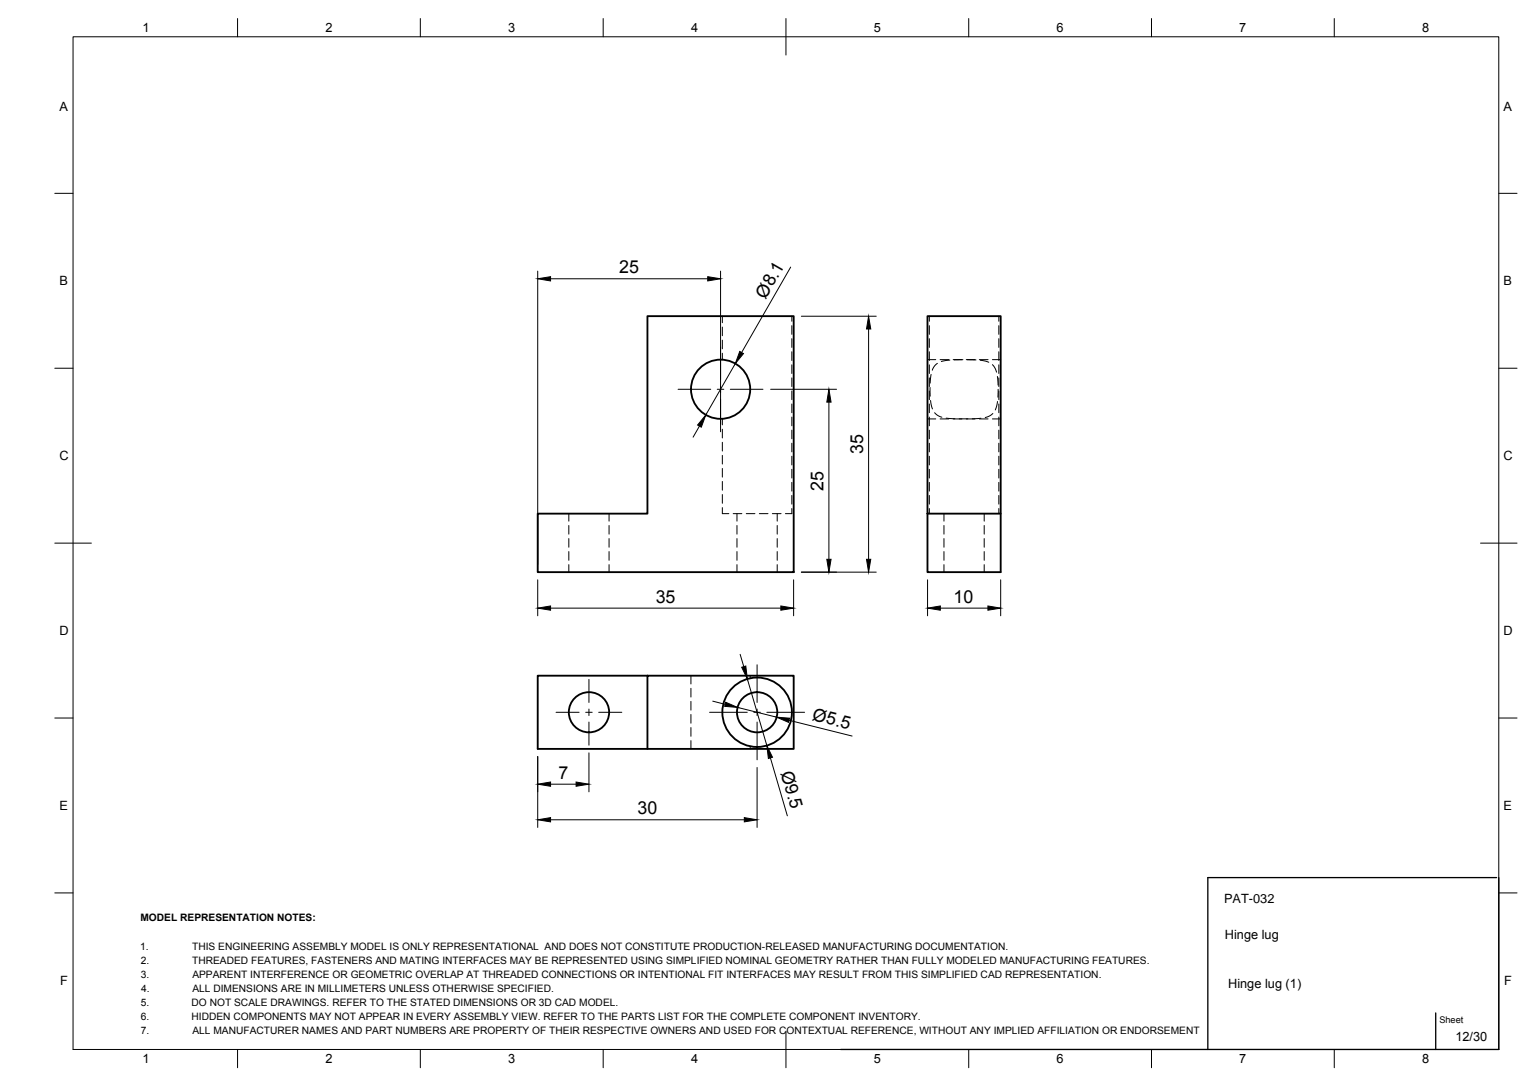
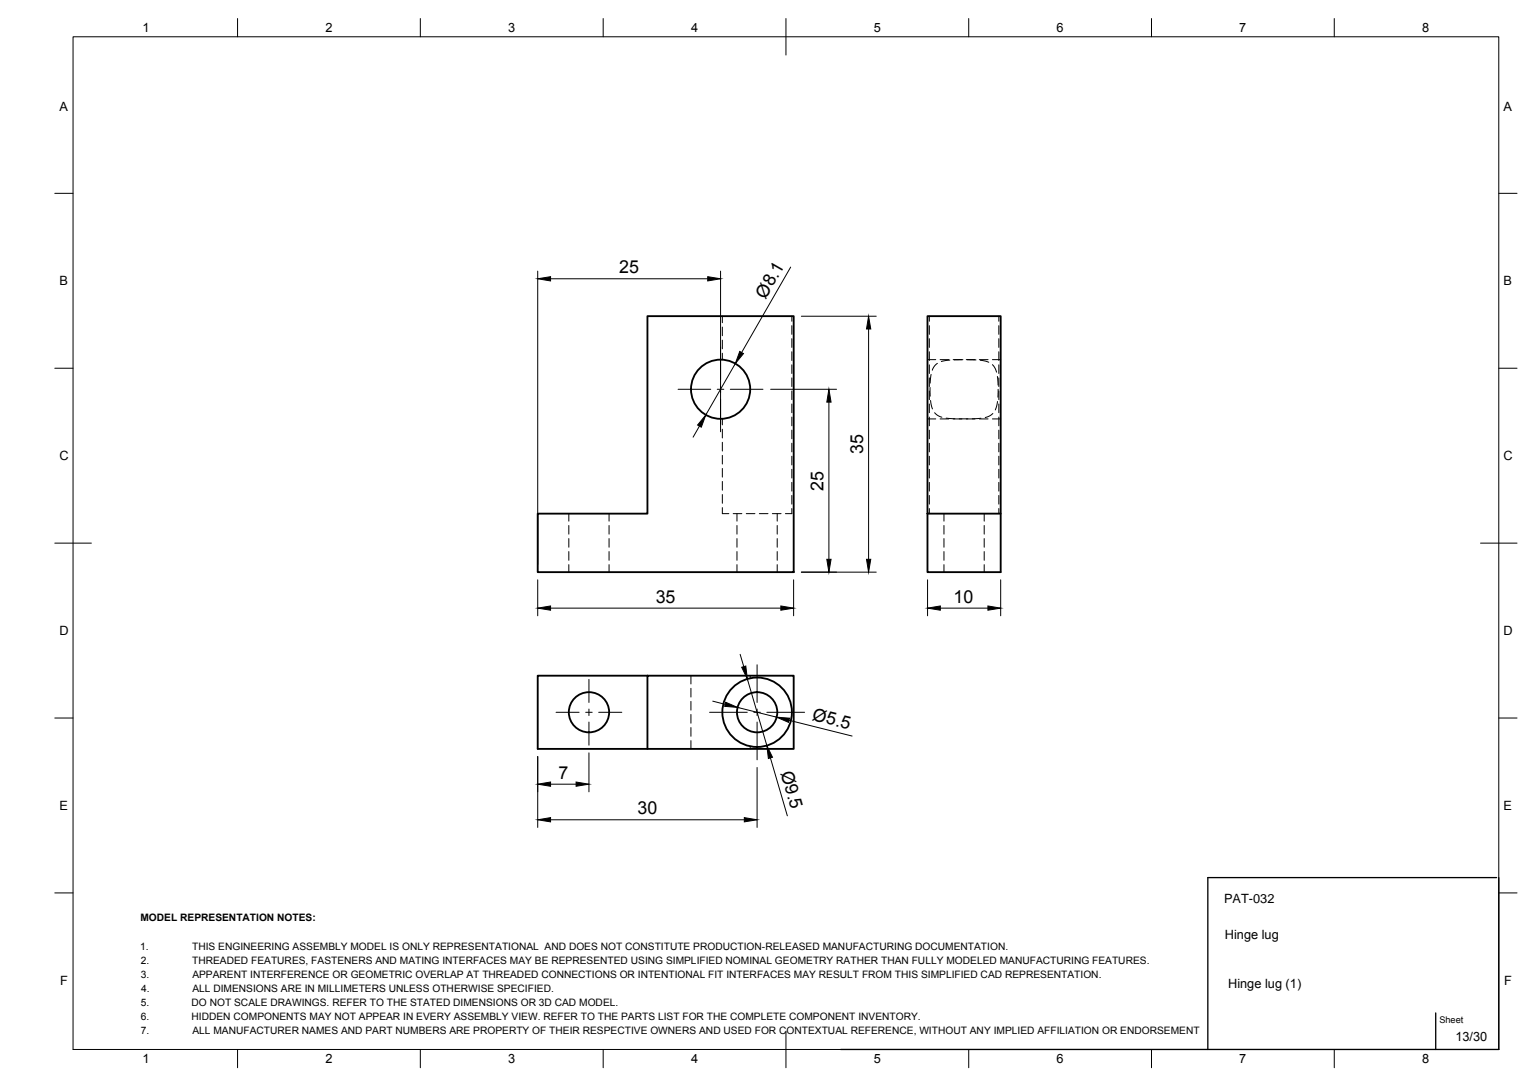
ISO-10303-21;
HEADER;
/* Generated by software containing ST-Developer
 * from STEP Tools, Inc. (www.steptools.com) 
 */

FILE_DESCRIPTION(
/* description */ ('Drill jig with bushing plate'),
/* implementation_level */ '2;1');

FILE_NAME(
/* name */ 'Hinge lug.step',
/* time_stamp */ '2026-10-27T10:51:08-07:00',
/* author */ (''),
/* organization */ (''),
/* preprocessor_version */ 'ST-DEVELOPER v20.2',
/* originating_system */ 'Autodesk Translation Framework v15.17.0.0',
/* authorisation */ '');

FILE_SCHEMA (('AUTOMOTIVE_DESIGN { 1 0 10303 214 3 1 1 }'));
ENDSEC;

DATA;
#10=MECHANICAL_DESIGN_GEOMETRIC_PRESENTATION_REPRESENTATION('',(#230),#6638);
#173=B_SPLINE_CURVE_WITH_KNOTS('',3,(#5774,#5775,#5776,#5777,#5778,#5779,
#5780,#5781,#5782,#5783,#5784,#5785,#5786,#5787,#5788,#5789,#5790,#5791,
#5792,#5793,#5794,#5795,#5796,#5797,#5798,#5799,#5800,#5801,#5802,#5803,
#5804,#5805,#5806,#5807,#5808,#5809,#5810,#5811,#5812,#5813,#5814,#5815,
#5816,#5817,#5818,#5819,#5820,#5821,#5822,#5823),.UNSPECIFIED.,.T.,.F.,
(4,2,2,2,2,2,2,2,2,2,2,2,2,2,2,2,2,2,2,2,2,2,2,2,4),(0.,0.177519856988816,
0.355039713977633,0.436196019741432,0.517352325505232,0.678532215702782,
0.839712105900332,1.00089199609788,1.16207188629543,1.24322819205923,1.32438449782303,
1.50190435481185,1.67942421180066,1.85694406878948,2.0344639257783,2.1156202315421,
2.1967765373059,2.35795642750345,2.519136317701,2.68031620789855,2.8414960980961,
2.9226524038599,3.0038087096237,3.18132856661251,3.35884842360133),
 .UNSPECIFIED.);
#182=SHAPE_REPRESENTATION_RELATIONSHIP('SRR','None',#6746,#206);
#206=ADVANCED_BREP_SHAPE_REPRESENTATION('',(#254),#6619);
#230=STYLED_ITEM('',(#6957),#254);
#254=MANIFOLD_SOLID_BREP('Body1',#3597);
#310=FACE_BOUND('',#818,.T.);
#311=FACE_BOUND('',#820,.T.);
#312=FACE_BOUND('',#824,.T.);
#313=FACE_BOUND('',#826,.T.);
#314=FACE_BOUND('',#829,.T.);
#315=FACE_BOUND('',#832,.T.);
#316=FACE_BOUND('',#833,.T.);
#317=FACE_BOUND('',#836,.T.);
#318=FACE_BOUND('',#838,.T.);
#405=PLANE('',#4007);
#406=PLANE('',#4017);
#407=PLANE('',#4018);
#408=PLANE('',#4019);
#409=PLANE('',#4020);
#410=PLANE('',#4021);
#411=PLANE('',#4022);
#412=PLANE('',#4023);
#413=PLANE('',#4024);
#562=FACE_OUTER_BOUND('',#817,.T.);
#563=FACE_OUTER_BOUND('',#819,.T.);
#564=FACE_OUTER_BOUND('',#821,.T.);
#565=FACE_OUTER_BOUND('',#822,.T.);
#566=FACE_OUTER_BOUND('',#823,.T.);
#567=FACE_OUTER_BOUND('',#825,.T.);
#568=FACE_OUTER_BOUND('',#827,.T.);
#569=FACE_OUTER_BOUND('',#828,.T.);
#570=FACE_OUTER_BOUND('',#830,.T.);
#571=FACE_OUTER_BOUND('',#831,.T.);
#572=FACE_OUTER_BOUND('',#834,.T.);
#573=FACE_OUTER_BOUND('',#835,.T.);
#574=FACE_OUTER_BOUND('',#837,.T.);
#817=EDGE_LOOP('',(#2689,#2690,#2691,#2692));
#818=EDGE_LOOP('',(#2693));
#819=EDGE_LOOP('',(#2694));
#820=EDGE_LOOP('',(#2695));
#821=EDGE_LOOP('',(#2696,#2697,#2698,#2699));
#822=EDGE_LOOP('',(#2700,#2701,#2702,#2703));
#823=EDGE_LOOP('',(#2704,#2705,#2706,#2707));
#824=EDGE_LOOP('',(#2708));
#825=EDGE_LOOP('',(#2709,#2710,#2711,#2712));
#826=EDGE_LOOP('',(#2713));
#827=EDGE_LOOP('',(#2714,#2715,#2716,#2717));
#828=EDGE_LOOP('',(#2718,#2719,#2720,#2721));
#829=EDGE_LOOP('',(#2722));
#830=EDGE_LOOP('',(#2723,#2724,#2725,#2726));
#831=EDGE_LOOP('',(#2727,#2728,#2729,#2730));
#832=EDGE_LOOP('',(#2731));
#833=EDGE_LOOP('',(#2732));
#834=EDGE_LOOP('',(#2733,#2734,#2735,#2736));
#835=EDGE_LOOP('',(#2737,#2738,#2739,#2740,#2741,#2742));
#836=EDGE_LOOP('',(#2743));
#837=EDGE_LOOP('',(#2744,#2745,#2746,#2747,#2748,#2749));
#838=EDGE_LOOP('',(#2750));
#1104=LINE('',#5771,#1365);
#1105=LINE('',#5830,#1366);
#1106=LINE('',#5835,#1367);
#1107=LINE('',#5841,#1368);
#1108=LINE('',#5846,#1369);
#1109=LINE('',#5848,#1370);
#1110=LINE('',#5850,#1371);
#1111=LINE('',#5851,#1372);
#1112=LINE('',#5854,#1373);
#1113=LINE('',#5856,#1374);
#1114=LINE('',#5857,#1375);
#1115=LINE('',#5860,#1376);
#1116=LINE('',#5862,#1377);
#1117=LINE('',#5863,#1378);
#1118=LINE('',#5866,#1379);
#1119=LINE('',#5868,#1380);
#1120=LINE('',#5869,#1381);
#1121=LINE('',#5872,#1382);
#1122=LINE('',#5874,#1383);
#1123=LINE('',#5875,#1384);
#1124=LINE('',#5877,#1385);
#1125=LINE('',#5878,#1386);
#1365=VECTOR('',#4653,0.475);
#1366=VECTOR('',#4664,0.275);
#1367=VECTOR('',#4669,0.275);
#1368=VECTOR('',#4676,0.405);
#1369=VECTOR('',#4681,1.);
#1370=VECTOR('',#4682,1.);
#1371=VECTOR('',#4683,1.);
#1372=VECTOR('',#4684,1.);
#1373=VECTOR('',#4687,1.);
#1374=VECTOR('',#4688,1.);
#1375=VECTOR('',#4689,1.);
#1376=VECTOR('',#4692,1.);
#1377=VECTOR('',#4693,1.);
#1378=VECTOR('',#4694,1.);
#1379=VECTOR('',#4697,1.);
#1380=VECTOR('',#4698,1.);
#1381=VECTOR('',#4699,1.);
#1382=VECTOR('',#4702,1.);
#1383=VECTOR('',#4703,1.);
#1384=VECTOR('',#4704,1.);
#1385=VECTOR('',#4707,1.);
#1386=VECTOR('',#4708,1.);
#1604=CIRCLE('',#4005,0.475);
#1605=CIRCLE('',#4006,0.475);
#1606=CIRCLE('',#4008,0.275);
#1607=CIRCLE('',#4010,0.275);
#1608=CIRCLE('',#4012,0.275);
#1609=CIRCLE('',#4013,0.275);
#1610=CIRCLE('',#4015,0.405);
#1611=CIRCLE('',#4016,0.405);
#1804=VERTEX_POINT('',#5768);
#1805=VERTEX_POINT('',#5770);
#1806=VERTEX_POINT('',#5773);
#1807=VERTEX_POINT('',#5825);
#1808=VERTEX_POINT('',#5828);
#1809=VERTEX_POINT('',#5832);
#1810=VERTEX_POINT('',#5834);
#1811=VERTEX_POINT('',#5838);
#1812=VERTEX_POINT('',#5840);
#1813=VERTEX_POINT('',#5844);
#1814=VERTEX_POINT('',#5845);
#1815=VERTEX_POINT('',#5847);
#1816=VERTEX_POINT('',#5849);
#1817=VERTEX_POINT('',#5853);
#1818=VERTEX_POINT('',#5855);
#1819=VERTEX_POINT('',#5859);
#1820=VERTEX_POINT('',#5861);
#1821=VERTEX_POINT('',#5865);
#1822=VERTEX_POINT('',#5867);
#1823=VERTEX_POINT('',#5871);
#1824=VERTEX_POINT('',#5873);
#2132=EDGE_CURVE('',#1804,#1804,#1604,.T.);
#2133=EDGE_CURVE('',#1804,#1805,#1104,.T.);
#2134=EDGE_CURVE('',#1805,#1805,#1605,.T.);
#2135=EDGE_CURVE('',#1806,#1806,#173,.T.);
#2136=EDGE_CURVE('',#1807,#1807,#1606,.T.);
#2137=EDGE_CURVE('',#1808,#1808,#1607,.T.);
#2138=EDGE_CURVE('',#1808,#1807,#1105,.T.);
#2139=EDGE_CURVE('',#1809,#1809,#1608,.T.);
#2140=EDGE_CURVE('',#1809,#1810,#1106,.T.);
#2141=EDGE_CURVE('',#1810,#1810,#1609,.T.);
#2142=EDGE_CURVE('',#1811,#1811,#1610,.T.);
#2143=EDGE_CURVE('',#1811,#1812,#1107,.T.);
#2144=EDGE_CURVE('',#1812,#1812,#1611,.T.);
#2145=EDGE_CURVE('',#1813,#1814,#1108,.T.);
#2146=EDGE_CURVE('',#1814,#1815,#1109,.T.);
#2147=EDGE_CURVE('',#1816,#1815,#1110,.T.);
#2148=EDGE_CURVE('',#1813,#1816,#1111,.T.);
#2149=EDGE_CURVE('',#1817,#1813,#1112,.T.);
#2150=EDGE_CURVE('',#1818,#1816,#1113,.T.);
#2151=EDGE_CURVE('',#1817,#1818,#1114,.T.);
#2152=EDGE_CURVE('',#1819,#1817,#1115,.T.);
#2153=EDGE_CURVE('',#1820,#1818,#1116,.T.);
#2154=EDGE_CURVE('',#1819,#1820,#1117,.T.);
#2155=EDGE_CURVE('',#1821,#1819,#1118,.T.);
#2156=EDGE_CURVE('',#1822,#1820,#1119,.T.);
#2157=EDGE_CURVE('',#1821,#1822,#1120,.T.);
#2158=EDGE_CURVE('',#1823,#1821,#1121,.T.);
#2159=EDGE_CURVE('',#1824,#1822,#1122,.T.);
#2160=EDGE_CURVE('',#1823,#1824,#1123,.T.);
#2161=EDGE_CURVE('',#1814,#1823,#1124,.T.);
#2162=EDGE_CURVE('',#1815,#1824,#1125,.T.);
#2689=ORIENTED_EDGE('',*,*,#2132,.F.);
#2690=ORIENTED_EDGE('',*,*,#2133,.T.);
#2691=ORIENTED_EDGE('',*,*,#2134,.F.);
#2692=ORIENTED_EDGE('',*,*,#2133,.F.);
#2693=ORIENTED_EDGE('',*,*,#2135,.F.);
#2694=ORIENTED_EDGE('',*,*,#2132,.T.);
#2695=ORIENTED_EDGE('',*,*,#2136,.F.);
#2696=ORIENTED_EDGE('',*,*,#2137,.F.);
#2697=ORIENTED_EDGE('',*,*,#2138,.T.);
#2698=ORIENTED_EDGE('',*,*,#2136,.T.);
#2699=ORIENTED_EDGE('',*,*,#2138,.F.);
#2700=ORIENTED_EDGE('',*,*,#2139,.F.);
#2701=ORIENTED_EDGE('',*,*,#2140,.T.);
#2702=ORIENTED_EDGE('',*,*,#2141,.F.);
#2703=ORIENTED_EDGE('',*,*,#2140,.F.);
#2704=ORIENTED_EDGE('',*,*,#2142,.F.);
#2705=ORIENTED_EDGE('',*,*,#2143,.T.);
#2706=ORIENTED_EDGE('',*,*,#2144,.F.);
#2707=ORIENTED_EDGE('',*,*,#2143,.F.);
#2708=ORIENTED_EDGE('',*,*,#2135,.T.);
#2709=ORIENTED_EDGE('',*,*,#2145,.T.);
#2710=ORIENTED_EDGE('',*,*,#2146,.T.);
#2711=ORIENTED_EDGE('',*,*,#2147,.F.);
#2712=ORIENTED_EDGE('',*,*,#2148,.F.);
#2713=ORIENTED_EDGE('',*,*,#2134,.T.);
#2714=ORIENTED_EDGE('',*,*,#2149,.T.);
#2715=ORIENTED_EDGE('',*,*,#2148,.T.);
#2716=ORIENTED_EDGE('',*,*,#2150,.F.);
#2717=ORIENTED_EDGE('',*,*,#2151,.F.);
#2718=ORIENTED_EDGE('',*,*,#2152,.T.);
#2719=ORIENTED_EDGE('',*,*,#2151,.T.);
#2720=ORIENTED_EDGE('',*,*,#2153,.F.);
#2721=ORIENTED_EDGE('',*,*,#2154,.F.);
#2722=ORIENTED_EDGE('',*,*,#2141,.T.);
#2723=ORIENTED_EDGE('',*,*,#2155,.T.);
#2724=ORIENTED_EDGE('',*,*,#2154,.T.);
#2725=ORIENTED_EDGE('',*,*,#2156,.F.);
#2726=ORIENTED_EDGE('',*,*,#2157,.F.);
#2727=ORIENTED_EDGE('',*,*,#2158,.T.);
#2728=ORIENTED_EDGE('',*,*,#2157,.T.);
#2729=ORIENTED_EDGE('',*,*,#2159,.F.);
#2730=ORIENTED_EDGE('',*,*,#2160,.F.);
#2731=ORIENTED_EDGE('',*,*,#2137,.T.);
#2732=ORIENTED_EDGE('',*,*,#2139,.T.);
#2733=ORIENTED_EDGE('',*,*,#2161,.T.);
#2734=ORIENTED_EDGE('',*,*,#2160,.T.);
#2735=ORIENTED_EDGE('',*,*,#2162,.F.);
#2736=ORIENTED_EDGE('',*,*,#2146,.F.);
#2737=ORIENTED_EDGE('',*,*,#2162,.T.);
#2738=ORIENTED_EDGE('',*,*,#2159,.T.);
#2739=ORIENTED_EDGE('',*,*,#2156,.T.);
#2740=ORIENTED_EDGE('',*,*,#2153,.T.);
#2741=ORIENTED_EDGE('',*,*,#2150,.T.);
#2742=ORIENTED_EDGE('',*,*,#2147,.T.);
#2743=ORIENTED_EDGE('',*,*,#2144,.T.);
#2744=ORIENTED_EDGE('',*,*,#2161,.F.);
#2745=ORIENTED_EDGE('',*,*,#2145,.F.);
#2746=ORIENTED_EDGE('',*,*,#2149,.F.);
#2747=ORIENTED_EDGE('',*,*,#2152,.F.);
#2748=ORIENTED_EDGE('',*,*,#2155,.F.);
#2749=ORIENTED_EDGE('',*,*,#2158,.F.);
#2750=ORIENTED_EDGE('',*,*,#2142,.T.);
#3325=CYLINDRICAL_SURFACE('',#4004,0.475);
#3326=CYLINDRICAL_SURFACE('',#4009,0.275);
#3327=CYLINDRICAL_SURFACE('',#4011,0.275);
#3328=CYLINDRICAL_SURFACE('',#4014,0.405);
#3437=ADVANCED_FACE('',(#562,#310),#3325,.F.);
#3438=ADVANCED_FACE('',(#563,#311),#405,.T.);
#3439=ADVANCED_FACE('',(#564),#3326,.F.);
#3440=ADVANCED_FACE('',(#565),#3327,.F.);
#3441=ADVANCED_FACE('',(#566,#312),#3328,.F.);
#3442=ADVANCED_FACE('',(#567,#313),#406,.T.);
#3443=ADVANCED_FACE('',(#568),#407,.T.);
#3444=ADVANCED_FACE('',(#569,#314),#408,.T.);
#3445=ADVANCED_FACE('',(#570),#409,.T.);
#3446=ADVANCED_FACE('',(#571,#315,#316),#410,.T.);
#3447=ADVANCED_FACE('',(#572),#411,.T.);
#3448=ADVANCED_FACE('',(#573,#317),#412,.T.);
#3449=ADVANCED_FACE('',(#574,#318),#413,.F.);
#3597=CLOSED_SHELL('',(#3437,#3438,#3439,#3440,#3441,#3442,#3443,#3444,
#3445,#3446,#3447,#3448,#3449));
#4003=AXIS2_PLACEMENT_3D('',#5766,#4647,#4648);
#4004=AXIS2_PLACEMENT_3D('',#5767,#4649,#4650);
#4005=AXIS2_PLACEMENT_3D('',#5769,#4651,#4652);
#4006=AXIS2_PLACEMENT_3D('',#5772,#4654,#4655);
#4007=AXIS2_PLACEMENT_3D('',#5824,#4656,#4657);
#4008=AXIS2_PLACEMENT_3D('',#5826,#4658,#4659);
#4009=AXIS2_PLACEMENT_3D('',#5827,#4660,#4661);
#4010=AXIS2_PLACEMENT_3D('',#5829,#4662,#4663);
#4011=AXIS2_PLACEMENT_3D('',#5831,#4665,#4666);
#4012=AXIS2_PLACEMENT_3D('',#5833,#4667,#4668);
#4013=AXIS2_PLACEMENT_3D('',#5836,#4670,#4671);
#4014=AXIS2_PLACEMENT_3D('',#5837,#4672,#4673);
#4015=AXIS2_PLACEMENT_3D('',#5839,#4674,#4675);
#4016=AXIS2_PLACEMENT_3D('',#5842,#4677,#4678);
#4017=AXIS2_PLACEMENT_3D('',#5843,#4679,#4680);
#4018=AXIS2_PLACEMENT_3D('',#5852,#4685,#4686);
#4019=AXIS2_PLACEMENT_3D('',#5858,#4690,#4691);
#4020=AXIS2_PLACEMENT_3D('',#5864,#4695,#4696);
#4021=AXIS2_PLACEMENT_3D('',#5870,#4700,#4701);
#4022=AXIS2_PLACEMENT_3D('',#5876,#4705,#4706);
#4023=AXIS2_PLACEMENT_3D('',#5879,#4709,#4710);
#4024=AXIS2_PLACEMENT_3D('',#5880,#4711,#4712);
#4647=DIRECTION('axis',(0.,0.,1.));
#4648=DIRECTION('refdir',(1.,0.,0.));
#4649=DIRECTION('center_axis',(0.,0.,1.));
#4650=DIRECTION('ref_axis',(1.,0.,0.));
#4651=DIRECTION('center_axis',(0.,0.,1.));
#4652=DIRECTION('ref_axis',(1.,0.,0.));
#4653=DIRECTION('',(0.,0.,1.));
#4654=DIRECTION('center_axis',(0.,0.,-1.));
#4655=DIRECTION('ref_axis',(1.,0.,0.));
#4656=DIRECTION('center_axis',(0.,0.,1.));
#4657=DIRECTION('ref_axis',(1.,0.,0.));
#4658=DIRECTION('center_axis',(0.,0.,1.));
#4659=DIRECTION('ref_axis',(1.,0.,0.));
#4660=DIRECTION('center_axis',(0.,0.,1.));
#4661=DIRECTION('ref_axis',(1.,0.,0.));
#4662=DIRECTION('center_axis',(0.,0.,1.));
#4663=DIRECTION('ref_axis',(1.,0.,0.));
#4664=DIRECTION('',(0.,0.,1.));
#4665=DIRECTION('center_axis',(0.,0.,1.));
#4666=DIRECTION('ref_axis',(1.,0.,0.));
#4667=DIRECTION('center_axis',(0.,0.,1.));
#4668=DIRECTION('ref_axis',(1.,0.,0.));
#4669=DIRECTION('',(0.,0.,1.));
#4670=DIRECTION('center_axis',(0.,0.,-1.));
#4671=DIRECTION('ref_axis',(1.,0.,0.));
#4672=DIRECTION('center_axis',(1.,0.,0.));
#4673=DIRECTION('ref_axis',(0.,0.,-1.));
#4674=DIRECTION('center_axis',(1.,0.,0.));
#4675=DIRECTION('ref_axis',(0.,0.,-1.));
#4676=DIRECTION('',(1.,0.,0.));
#4677=DIRECTION('center_axis',(-1.,0.,0.));
#4678=DIRECTION('ref_axis',(0.,0.,-1.));
#4679=DIRECTION('center_axis',(0.,0.,1.));
#4680=DIRECTION('ref_axis',(0.,-1.,0.));
#4681=DIRECTION('',(0.,-1.,0.));
#4682=DIRECTION('',(1.,0.,0.));
#4683=DIRECTION('',(0.,-1.,0.));
#4684=DIRECTION('',(1.,0.,0.));
#4685=DIRECTION('center_axis',(0.,1.,0.));
#4686=DIRECTION('ref_axis',(0.,0.,1.));
#4687=DIRECTION('',(0.,0.,1.));
#4688=DIRECTION('',(0.,0.,1.));
#4689=DIRECTION('',(1.,0.,0.));
#4690=DIRECTION('center_axis',(0.,0.,1.));
#4691=DIRECTION('ref_axis',(0.,-1.,0.));
#4692=DIRECTION('',(0.,-1.,0.));
#4693=DIRECTION('',(0.,-1.,0.));
#4694=DIRECTION('',(1.,0.,0.));
#4695=DIRECTION('center_axis',(0.,1.,0.));
#4696=DIRECTION('ref_axis',(0.,0.,1.));
#4697=DIRECTION('',(0.,0.,1.));
#4698=DIRECTION('',(0.,0.,1.));
#4699=DIRECTION('',(1.,0.,0.));
#4700=DIRECTION('center_axis',(0.,0.,-1.));
#4701=DIRECTION('ref_axis',(0.,1.,0.));
#4702=DIRECTION('',(0.,1.,0.));
#4703=DIRECTION('',(0.,1.,0.));
#4704=DIRECTION('',(1.,0.,0.));
#4705=DIRECTION('center_axis',(0.,-1.,0.));
#4706=DIRECTION('ref_axis',(0.,0.,-1.));
#4707=DIRECTION('',(0.,0.,-1.));
#4708=DIRECTION('',(0.,0.,-1.));
#4709=DIRECTION('center_axis',(1.,0.,0.));
#4710=DIRECTION('ref_axis',(0.,0.,-1.));
#4711=DIRECTION('center_axis',(1.,0.,0.));
#4712=DIRECTION('ref_axis',(0.,0.,-1.));
#5766=CARTESIAN_POINT('',(0.,0.,0.));
#5767=CARTESIAN_POINT('Origin',(-6.5,-6.5,1.8));
#5768=CARTESIAN_POINT('',(-6.975,-6.5,1.8));
#5769=CARTESIAN_POINT('Origin',(-6.5,-6.5,1.8));
#5770=CARTESIAN_POINT('',(-6.975,-6.5,4.5));
#5771=CARTESIAN_POINT('',(-6.975,-6.5,1.8));
#5772=CARTESIAN_POINT('Origin',(-6.5,-6.5,4.5));
#5773=CARTESIAN_POINT('',(-6.9654030511288,-6.405,3.5));
#5774=CARTESIAN_POINT('Ctrl Pts',(-6.9654030511288,-6.405,3.5));
#5775=CARTESIAN_POINT('Ctrl Pts',(-6.9654030511288,-6.405,3.44082671433706));
#5776=CARTESIAN_POINT('Ctrl Pts',(-6.96319194510978,-6.391162819218,3.3786038562345));
#5777=CARTESIAN_POINT('Ctrl Pts',(-6.9474004570938,-6.33805779261652,3.26878119899199));
#5778=CARTESIAN_POINT('Ctrl Pts',(-6.93296763252909,-6.29875591394082,3.22132213181236));
#5779=CARTESIAN_POINT('Ctrl Pts',(-6.89697744222372,-6.23823300006139,3.17155768103299));
#5780=CARTESIAN_POINT('Ctrl Pts',(-6.88237408148839,-6.2169021926909,3.15715697182391));
#5781=CARTESIAN_POINT('Ctrl Pts',(-6.84782319019902,-6.17538739566531,3.13417605500228));
#5782=CARTESIAN_POINT('Ctrl Pts',(-6.8278469830262,-6.1552757719279,3.12550838237099));
#5783=CARTESIAN_POINT('Ctrl Pts',(-6.76795622589237,-6.10432382827604,3.1070097286502));
#5784=CARTESIAN_POINT('Ctrl Pts',(-6.71846870594364,-6.07437258197005,3.10138466314703));
#5785=CARTESIAN_POINT('Ctrl Pts',(-6.61134072173687,-6.03471454832095,3.09599463066268));
#5786=CARTESIAN_POINT('Ctrl Pts',(-6.55372663006585,-6.025,3.09577234137185));
#5787=CARTESIAN_POINT('Ctrl Pts',(-6.44627336993415,-6.025,3.09577234137185));
#5788=CARTESIAN_POINT('Ctrl Pts',(-6.38865927826313,-6.03471454832095,3.09599463066268));
#5789=CARTESIAN_POINT('Ctrl Pts',(-6.28153129405636,-6.07437258197005,3.10138466314702));
#5790=CARTESIAN_POINT('Ctrl Pts',(-6.23204377410763,-6.10432382827604,3.1070097286502));
#5791=CARTESIAN_POINT('Ctrl Pts',(-6.1721530169738,-6.1552757719279,3.12550838237099));
#5792=CARTESIAN_POINT('Ctrl Pts',(-6.15217680980098,-6.17538739566531,3.13417605500228));
#5793=CARTESIAN_POINT('Ctrl Pts',(-6.11762591851161,-6.2169021926909,3.15715697182391));
#5794=CARTESIAN_POINT('Ctrl Pts',(-6.10302255777628,-6.23823300006139,3.17155768103299));
#5795=CARTESIAN_POINT('Ctrl Pts',(-6.06703236747091,-6.29875591394082,3.22132213181236));
#5796=CARTESIAN_POINT('Ctrl Pts',(-6.0525995429062,-6.33805779261652,3.26878119899199));
#5797=CARTESIAN_POINT('Ctrl Pts',(-6.03680805489022,-6.391162819218,3.3786038562345));
#5798=CARTESIAN_POINT('Ctrl Pts',(-6.0345969488712,-6.405,3.44082671433706));
#5799=CARTESIAN_POINT('Ctrl Pts',(-6.0345969488712,-6.405,3.55917328566294));
#5800=CARTESIAN_POINT('Ctrl Pts',(-6.03680805489022,-6.391162819218,3.6213961437655));
#5801=CARTESIAN_POINT('Ctrl Pts',(-6.0525995429062,-6.33805779261652,3.73121880100801));
#5802=CARTESIAN_POINT('Ctrl Pts',(-6.06703236747091,-6.29875591394082,3.77867786818764));
#5803=CARTESIAN_POINT('Ctrl Pts',(-6.10302255777628,-6.23823300006139,3.82844231896701));
#5804=CARTESIAN_POINT('Ctrl Pts',(-6.1176259185116,-6.2169021926909,3.84284302817609));
#5805=CARTESIAN_POINT('Ctrl Pts',(-6.15217680980098,-6.17538739566531,3.86582394499772));
#5806=CARTESIAN_POINT('Ctrl Pts',(-6.1721530169738,-6.1552757719279,3.87449161762901));
#5807=CARTESIAN_POINT('Ctrl Pts',(-6.23204377410763,-6.10432382827604,3.8929902713498));
#5808=CARTESIAN_POINT('Ctrl Pts',(-6.28153129405636,-6.07437258197005,3.89861533685297));
#5809=CARTESIAN_POINT('Ctrl Pts',(-6.38865927826313,-6.03471454832095,3.90400536933732));
#5810=CARTESIAN_POINT('Ctrl Pts',(-6.44627336993415,-6.025,3.90422765862815));
#5811=CARTESIAN_POINT('Ctrl Pts',(-6.55372663006585,-6.025,3.90422765862815));
#5812=CARTESIAN_POINT('Ctrl Pts',(-6.61134072173687,-6.03471454832095,3.90400536933732));
#5813=CARTESIAN_POINT('Ctrl Pts',(-6.71846870594364,-6.07437258197005,3.89861533685297));
#5814=CARTESIAN_POINT('Ctrl Pts',(-6.76795622589237,-6.10432382827604,3.8929902713498));
#5815=CARTESIAN_POINT('Ctrl Pts',(-6.8278469830262,-6.1552757719279,3.87449161762901));
#5816=CARTESIAN_POINT('Ctrl Pts',(-6.84782319019902,-6.17538739566531,3.86582394499772));
#5817=CARTESIAN_POINT('Ctrl Pts',(-6.8823740814884,-6.21690219269089,3.84284302817609));
#5818=CARTESIAN_POINT('Ctrl Pts',(-6.89697744222372,-6.23823300006139,3.82844231896701));
#5819=CARTESIAN_POINT('Ctrl Pts',(-6.93296763252909,-6.29875591394082,3.77867786818764));
#5820=CARTESIAN_POINT('Ctrl Pts',(-6.9474004570938,-6.33805779261652,3.73121880100801));
#5821=CARTESIAN_POINT('Ctrl Pts',(-6.96319194510978,-6.391162819218,3.6213961437655));
#5822=CARTESIAN_POINT('Ctrl Pts',(-6.9654030511288,-6.405,3.55917328566294));
#5823=CARTESIAN_POINT('Ctrl Pts',(-6.9654030511288,-6.405,3.5));
#5824=CARTESIAN_POINT('Origin',(-6.5,-6.5,1.8));
#5825=CARTESIAN_POINT('',(-6.775,-6.5,1.8));
#5826=CARTESIAN_POINT('Origin',(-6.5,-6.5,1.8));
#5827=CARTESIAN_POINT('Origin',(-6.5,-6.5,0.9));
#5828=CARTESIAN_POINT('',(-6.775,-6.5,1.));
#5829=CARTESIAN_POINT('Origin',(-6.5,-6.5,1.));
#5830=CARTESIAN_POINT('',(-6.775,-6.5,0.9));
#5831=CARTESIAN_POINT('Origin',(-6.5,-4.2,0.9));
#5832=CARTESIAN_POINT('',(-6.775,-4.2,1.));
#5833=CARTESIAN_POINT('Origin',(-6.5,-4.2,1.));
#5834=CARTESIAN_POINT('',(-6.775,-4.2,1.8));
#5835=CARTESIAN_POINT('',(-6.775,-4.2,0.9));
#5836=CARTESIAN_POINT('Origin',(-6.5,-4.2,1.8));
#5837=CARTESIAN_POINT('Origin',(-7.1,-6.,3.5));
#5838=CARTESIAN_POINT('',(-7.,-6.,3.905));
#5839=CARTESIAN_POINT('Origin',(-7.,-6.,3.5));
#5840=CARTESIAN_POINT('',(-6.,-6.,3.905));
#5841=CARTESIAN_POINT('',(-7.1,-6.,3.905));
#5842=CARTESIAN_POINT('Origin',(-6.,-6.,3.5));
#5843=CARTESIAN_POINT('Origin',(-7.,-5.,4.5));
#5844=CARTESIAN_POINT('',(-7.,-5.,4.5));
#5845=CARTESIAN_POINT('',(-7.,-7.,4.5));
#5846=CARTESIAN_POINT('',(-7.,-5.,4.5));
#5847=CARTESIAN_POINT('',(-6.,-7.,4.5));
#5848=CARTESIAN_POINT('',(-7.,-7.,4.5));
#5849=CARTESIAN_POINT('',(-6.,-5.,4.5));
#5850=CARTESIAN_POINT('',(-6.,-5.,4.5));
#5851=CARTESIAN_POINT('',(-7.,-5.,4.5));
#5852=CARTESIAN_POINT('Origin',(-7.,-5.,1.8));
#5853=CARTESIAN_POINT('',(-7.,-5.,1.8));
#5854=CARTESIAN_POINT('',(-7.,-5.,1.8));
#5855=CARTESIAN_POINT('',(-6.,-5.,1.8));
#5856=CARTESIAN_POINT('',(-6.,-5.,1.8));
#5857=CARTESIAN_POINT('',(-7.,-5.,1.8));
#5858=CARTESIAN_POINT('Origin',(-7.,-3.5,1.8));
#5859=CARTESIAN_POINT('',(-7.,-3.5,1.8));
#5860=CARTESIAN_POINT('',(-7.,-3.5,1.8));
#5861=CARTESIAN_POINT('',(-6.,-3.5,1.8));
#5862=CARTESIAN_POINT('',(-6.,-3.5,1.8));
#5863=CARTESIAN_POINT('',(-7.,-3.5,1.8));
#5864=CARTESIAN_POINT('Origin',(-7.,-3.5,1.));
#5865=CARTESIAN_POINT('',(-7.,-3.5,1.));
#5866=CARTESIAN_POINT('',(-7.,-3.5,1.));
#5867=CARTESIAN_POINT('',(-6.,-3.5,1.));
#5868=CARTESIAN_POINT('',(-6.,-3.5,1.));
#5869=CARTESIAN_POINT('',(-7.,-3.5,1.));
#5870=CARTESIAN_POINT('Origin',(-7.,-7.,1.));
#5871=CARTESIAN_POINT('',(-7.,-7.,1.));
#5872=CARTESIAN_POINT('',(-7.,-7.,1.));
#5873=CARTESIAN_POINT('',(-6.,-7.,1.));
#5874=CARTESIAN_POINT('',(-6.,-7.,1.));
#5875=CARTESIAN_POINT('',(-7.,-7.,1.));
#5876=CARTESIAN_POINT('Origin',(-7.,-7.,4.5));
#5877=CARTESIAN_POINT('',(-7.,-7.,4.5));
#5878=CARTESIAN_POINT('',(-6.,-7.,4.5));
#5879=CARTESIAN_POINT('Origin',(-6.,-5.25,2.75));
#5880=CARTESIAN_POINT('Origin',(-7.,-5.25,2.75));
#6590=UNCERTAINTY_MEASURE_WITH_UNIT(LENGTH_MEASURE(0.001),#6639,
'DISTANCE_ACCURACY_VALUE',
'Maximum model space distance between geometric entities at asserted c
onnectivities');
#6609=UNCERTAINTY_MEASURE_WITH_UNIT(LENGTH_MEASURE(0.001),#6639,
'DISTANCE_ACCURACY_VALUE',
'Maximum model space distance between geometric entities at asserted c
onnectivities');
#6619=(
GEOMETRIC_REPRESENTATION_CONTEXT(3)
GLOBAL_UNCERTAINTY_ASSIGNED_CONTEXT((#6590))
GLOBAL_UNIT_ASSIGNED_CONTEXT((#6639,#6641,#6642))
REPRESENTATION_CONTEXT('','3D')
);
#6638=(
GEOMETRIC_REPRESENTATION_CONTEXT(3)
GLOBAL_UNCERTAINTY_ASSIGNED_CONTEXT((#6609))
GLOBAL_UNIT_ASSIGNED_CONTEXT((#6639,#6641,#6642))
REPRESENTATION_CONTEXT('','3D')
);
#6639=(
LENGTH_UNIT()
NAMED_UNIT(*)
SI_UNIT(.CENTI.,.METRE.)
);
#6641=(
NAMED_UNIT(*)
PLANE_ANGLE_UNIT()
SI_UNIT($,.RADIAN.)
);
#6642=(
NAMED_UNIT(*)
SI_UNIT($,.STERADIAN.)
SOLID_ANGLE_UNIT()
);
#6652=SHAPE_DEFINITION_REPRESENTATION(#6680,#6746);
#6680=PRODUCT_DEFINITION_SHAPE('',$,#6775);
#6746=SHAPE_REPRESENTATION('',(#4003),#6619);
#6765=PRODUCT_DEFINITION_CONTEXT('part definition',#6851,'design');
#6775=PRODUCT_DEFINITION('Hinge lug','Hinge lug',#6803,#6765);
#6803=PRODUCT_DEFINITION_FORMATION('',$,#6862);
#6851=APPLICATION_CONTEXT(
'Core Data for Automotive Mechanical Design Process');
#6852=PRODUCT_CONTEXT('part definition',#6851,'mechanical');
#6862=PRODUCT('Hinge lug','Hinge lug','Hinge lug',(#6852));
#6951=COLOUR_RGB('Off White',0.89,0.88,0.83);
#6952=FILL_AREA_STYLE_COLOUR('',#6951);
#6953=FILL_AREA_STYLE('',(#6952));
#6954=SURFACE_STYLE_FILL_AREA(#6953);
#6955=SURFACE_SIDE_STYLE('',(#6954));
#6956=SURFACE_STYLE_USAGE(.BOTH.,#6955);
#6957=PRESENTATION_STYLE_ASSIGNMENT((#6956));
ENDSEC;
END-ISO-10303-21;
